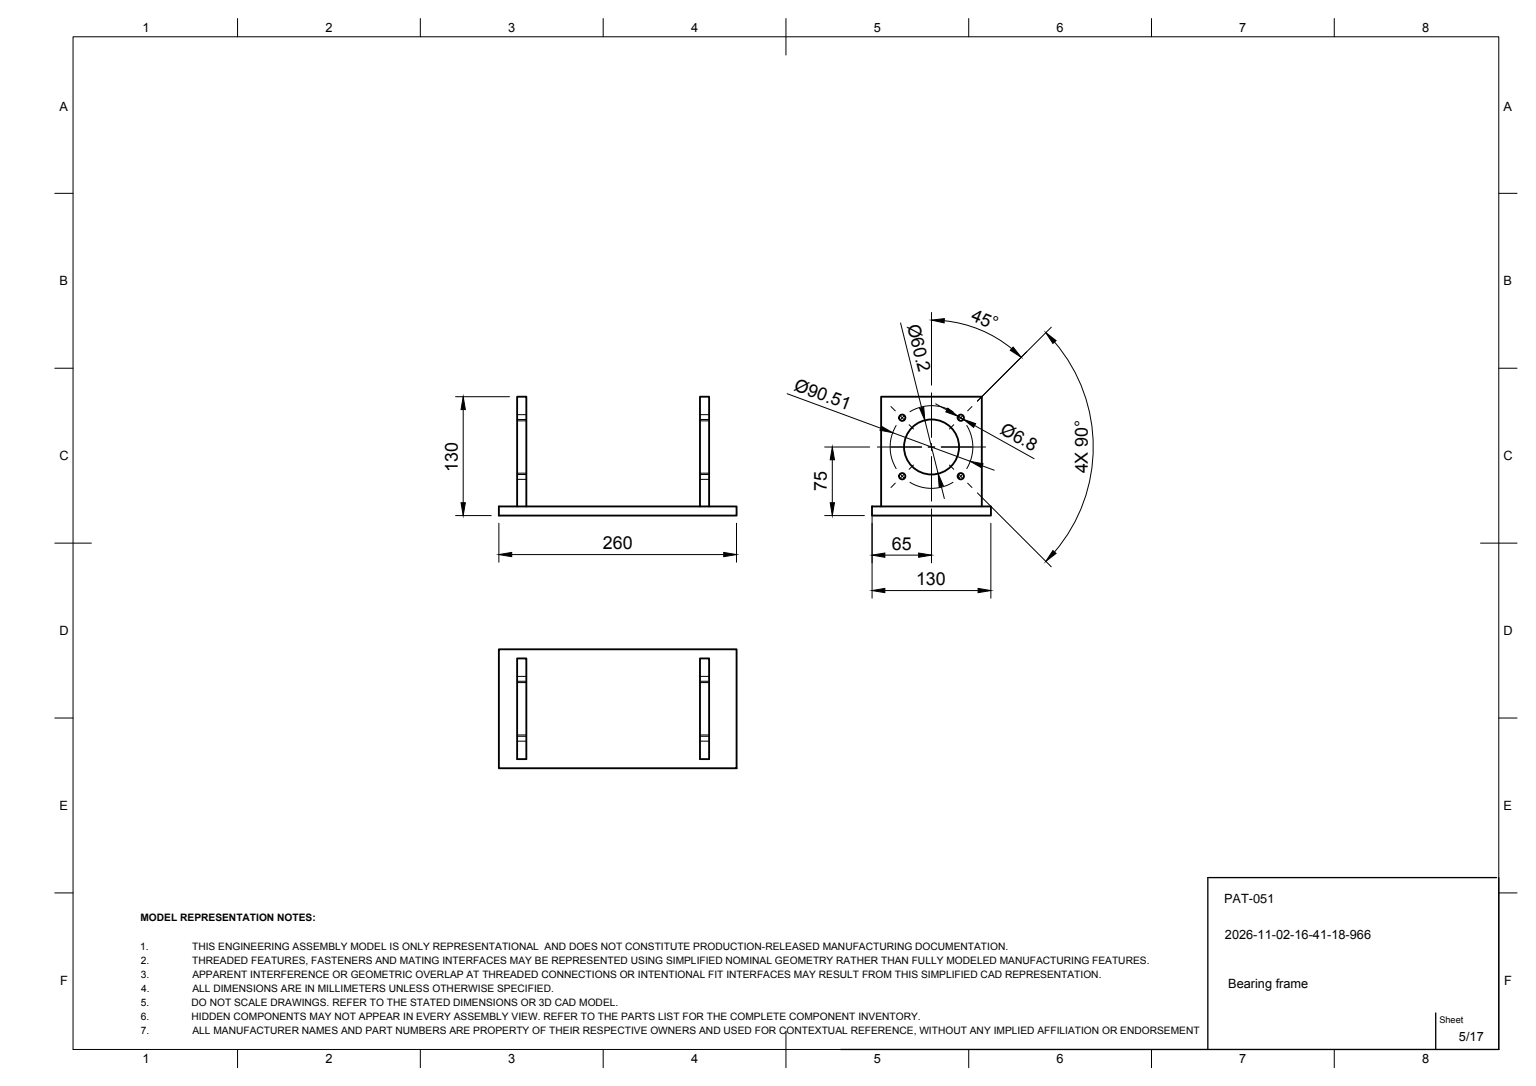
ISO-10303-21;
HEADER;
/* Generated by software containing ST-Developer
 * from STEP Tools, Inc. (www.steptools.com) 
 */

FILE_DESCRIPTION(
/* description */ ('Hand-crank flanged shaft unit'),
/* implementation_level */ '2;1');

FILE_NAME(
/* name */ 'Bearing frame.step',
/* time_stamp */ '2026-10-27T18:35:45-07:00',
/* author */ (''),
/* organization */ (''),
/* preprocessor_version */ 'ST-DEVELOPER v20.2',
/* originating_system */ 'Autodesk Translation Framework v15.17.0.0',
/* authorisation */ '');

FILE_SCHEMA (('AUTOMOTIVE_DESIGN { 1 0 10303 214 3 1 1 }'));
ENDSEC;

DATA;
#10=MECHANICAL_DESIGN_GEOMETRIC_PRESENTATION_REPRESENTATION('',(#279),#6805);
#239=SHAPE_REPRESENTATION_RELATIONSHIP('SRR','None',#6900,#259);
#259=ADVANCED_BREP_SHAPE_REPRESENTATION('',(#300),#6783);
#279=STYLED_ITEM('',(#7091),#300);
#300=MANIFOLD_SOLID_BREP('Body1',#3320);
#320=FACE_BOUND('',#712,.T.);
#321=FACE_BOUND('',#713,.T.);
#322=FACE_BOUND('',#714,.T.);
#323=FACE_BOUND('',#715,.T.);
#324=FACE_BOUND('',#716,.T.);
#325=FACE_BOUND('',#718,.T.);
#326=FACE_BOUND('',#719,.T.);
#327=FACE_BOUND('',#720,.T.);
#328=FACE_BOUND('',#721,.T.);
#329=FACE_BOUND('',#722,.T.);
#330=FACE_BOUND('',#732,.T.);
#331=FACE_BOUND('',#733,.T.);
#332=FACE_BOUND('',#734,.T.);
#333=FACE_BOUND('',#735,.T.);
#334=FACE_BOUND('',#736,.T.);
#335=FACE_BOUND('',#738,.T.);
#336=FACE_BOUND('',#739,.T.);
#337=FACE_BOUND('',#740,.T.);
#338=FACE_BOUND('',#741,.T.);
#339=FACE_BOUND('',#742,.T.);
#340=FACE_BOUND('',#748,.T.);
#341=FACE_BOUND('',#749,.T.);
#410=PLANE('',#3570);
#411=PLANE('',#3571);
#412=PLANE('',#3572);
#413=PLANE('',#3573);
#414=PLANE('',#3574);
#415=PLANE('',#3590);
#416=PLANE('',#3591);
#417=PLANE('',#3592);
#418=PLANE('',#3593);
#419=PLANE('',#3594);
#420=PLANE('',#3595);
#421=PLANE('',#3596);
#422=PLANE('',#3597);
#423=PLANE('',#3598);
#424=PLANE('',#3599);
#425=PLANE('',#3600);
#515=FACE_OUTER_BOUND('',#703,.T.);
#516=FACE_OUTER_BOUND('',#704,.T.);
#517=FACE_OUTER_BOUND('',#705,.T.);
#518=FACE_OUTER_BOUND('',#706,.T.);
#519=FACE_OUTER_BOUND('',#707,.T.);
#520=FACE_OUTER_BOUND('',#708,.T.);
#521=FACE_OUTER_BOUND('',#709,.T.);
#522=FACE_OUTER_BOUND('',#710,.T.);
#523=FACE_OUTER_BOUND('',#711,.T.);
#524=FACE_OUTER_BOUND('',#717,.T.);
#525=FACE_OUTER_BOUND('',#723,.T.);
#526=FACE_OUTER_BOUND('',#724,.T.);
#527=FACE_OUTER_BOUND('',#725,.T.);
#528=FACE_OUTER_BOUND('',#726,.T.);
#529=FACE_OUTER_BOUND('',#727,.T.);
#530=FACE_OUTER_BOUND('',#728,.T.);
#531=FACE_OUTER_BOUND('',#729,.T.);
#532=FACE_OUTER_BOUND('',#730,.T.);
#533=FACE_OUTER_BOUND('',#731,.T.);
#534=FACE_OUTER_BOUND('',#737,.T.);
#535=FACE_OUTER_BOUND('',#743,.T.);
#536=FACE_OUTER_BOUND('',#744,.T.);
#537=FACE_OUTER_BOUND('',#745,.T.);
#538=FACE_OUTER_BOUND('',#746,.T.);
#539=FACE_OUTER_BOUND('',#747,.T.);
#540=FACE_OUTER_BOUND('',#750,.T.);
#703=EDGE_LOOP('',(#2251,#2252,#2253,#2254));
#704=EDGE_LOOP('',(#2255,#2256,#2257,#2258));
#705=EDGE_LOOP('',(#2259,#2260,#2261,#2262));
#706=EDGE_LOOP('',(#2263,#2264,#2265,#2266));
#707=EDGE_LOOP('',(#2267,#2268,#2269,#2270));
#708=EDGE_LOOP('',(#2271,#2272,#2273,#2274));
#709=EDGE_LOOP('',(#2275,#2276,#2277,#2278));
#710=EDGE_LOOP('',(#2279,#2280,#2281,#2282));
#711=EDGE_LOOP('',(#2283,#2284,#2285,#2286));
#712=EDGE_LOOP('',(#2287));
#713=EDGE_LOOP('',(#2288));
#714=EDGE_LOOP('',(#2289));
#715=EDGE_LOOP('',(#2290));
#716=EDGE_LOOP('',(#2291));
#717=EDGE_LOOP('',(#2292,#2293,#2294,#2295));
#718=EDGE_LOOP('',(#2296));
#719=EDGE_LOOP('',(#2297));
#720=EDGE_LOOP('',(#2298));
#721=EDGE_LOOP('',(#2299));
#722=EDGE_LOOP('',(#2300));
#723=EDGE_LOOP('',(#2301,#2302,#2303,#2304));
#724=EDGE_LOOP('',(#2305,#2306,#2307,#2308));
#725=EDGE_LOOP('',(#2309,#2310,#2311,#2312));
#726=EDGE_LOOP('',(#2313,#2314,#2315,#2316));
#727=EDGE_LOOP('',(#2317,#2318,#2319,#2320));
#728=EDGE_LOOP('',(#2321,#2322,#2323,#2324));
#729=EDGE_LOOP('',(#2325,#2326,#2327,#2328));
#730=EDGE_LOOP('',(#2329,#2330,#2331,#2332));
#731=EDGE_LOOP('',(#2333,#2334,#2335,#2336));
#732=EDGE_LOOP('',(#2337));
#733=EDGE_LOOP('',(#2338));
#734=EDGE_LOOP('',(#2339));
#735=EDGE_LOOP('',(#2340));
#736=EDGE_LOOP('',(#2341));
#737=EDGE_LOOP('',(#2342,#2343,#2344,#2345));
#738=EDGE_LOOP('',(#2346));
#739=EDGE_LOOP('',(#2347));
#740=EDGE_LOOP('',(#2348));
#741=EDGE_LOOP('',(#2349));
#742=EDGE_LOOP('',(#2350));
#743=EDGE_LOOP('',(#2351,#2352,#2353,#2354));
#744=EDGE_LOOP('',(#2355,#2356,#2357,#2358));
#745=EDGE_LOOP('',(#2359,#2360,#2361,#2362));
#746=EDGE_LOOP('',(#2363,#2364,#2365,#2366));
#747=EDGE_LOOP('',(#2367,#2368,#2369,#2370));
#748=EDGE_LOOP('',(#2371,#2372,#2373,#2374));
#749=EDGE_LOOP('',(#2375,#2376,#2377,#2378));
#750=EDGE_LOOP('',(#2379,#2380,#2381,#2382));
#981=LINE('',#4939,#1209);
#982=LINE('',#4945,#1210);
#983=LINE('',#4951,#1211);
#984=LINE('',#4957,#1212);
#985=LINE('',#4963,#1213);
#986=LINE('',#4968,#1214);
#987=LINE('',#4970,#1215);
#988=LINE('',#4972,#1216);
#989=LINE('',#4973,#1217);
#990=LINE('',#4977,#1218);
#991=LINE('',#4979,#1219);
#992=LINE('',#4981,#1220);
#993=LINE('',#4982,#1221);
#994=LINE('',#4984,#1222);
#995=LINE('',#4985,#1223);
#996=LINE('',#4987,#1224);
#997=LINE('',#4989,#1225);
#998=LINE('',#4994,#1226);
#999=LINE('',#5000,#1227);
#1000=LINE('',#5006,#1228);
#1001=LINE('',#5012,#1229);
#1002=LINE('',#5018,#1230);
#1003=LINE('',#5023,#1231);
#1004=LINE('',#5025,#1232);
#1005=LINE('',#5027,#1233);
#1006=LINE('',#5028,#1234);
#1007=LINE('',#5032,#1235);
#1008=LINE('',#5034,#1236);
#1009=LINE('',#5036,#1237);
#1010=LINE('',#5037,#1238);
#1011=LINE('',#5039,#1239);
#1012=LINE('',#5040,#1240);
#1013=LINE('',#5042,#1241);
#1014=LINE('',#5044,#1242);
#1015=LINE('',#5048,#1243);
#1016=LINE('',#5050,#1244);
#1017=LINE('',#5052,#1245);
#1018=LINE('',#5053,#1246);
#1019=LINE('',#5056,#1247);
#1020=LINE('',#5058,#1248);
#1021=LINE('',#5059,#1249);
#1022=LINE('',#5062,#1250);
#1023=LINE('',#5064,#1251);
#1024=LINE('',#5065,#1252);
#1025=LINE('',#5067,#1253);
#1026=LINE('',#5068,#1254);
#1209=VECTOR('',#3946,0.34);
#1210=VECTOR('',#3953,0.34);
#1211=VECTOR('',#3960,0.34);
#1212=VECTOR('',#3967,0.34);
#1213=VECTOR('',#3974,3.01);
#1214=VECTOR('',#3979,1.);
#1215=VECTOR('',#3980,1.);
#1216=VECTOR('',#3981,1.);
#1217=VECTOR('',#3982,1.);
#1218=VECTOR('',#3985,1.);
#1219=VECTOR('',#3986,1.);
#1220=VECTOR('',#3987,1.);
#1221=VECTOR('',#3988,1.);
#1222=VECTOR('',#3991,1.);
#1223=VECTOR('',#3992,1.);
#1224=VECTOR('',#3995,1.);
#1225=VECTOR('',#3998,1.);
#1226=VECTOR('',#4003,0.34);
#1227=VECTOR('',#4010,0.34);
#1228=VECTOR('',#4017,0.34);
#1229=VECTOR('',#4024,0.34);
#1230=VECTOR('',#4031,3.01);
#1231=VECTOR('',#4036,1.);
#1232=VECTOR('',#4037,1.);
#1233=VECTOR('',#4038,1.);
#1234=VECTOR('',#4039,1.);
#1235=VECTOR('',#4042,1.);
#1236=VECTOR('',#4043,1.);
#1237=VECTOR('',#4044,1.);
#1238=VECTOR('',#4045,1.);
#1239=VECTOR('',#4048,1.);
#1240=VECTOR('',#4049,1.);
#1241=VECTOR('',#4052,1.);
#1242=VECTOR('',#4055,1.);
#1243=VECTOR('',#4058,1.);
#1244=VECTOR('',#4059,1.);
#1245=VECTOR('',#4060,1.);
#1246=VECTOR('',#4061,1.);
#1247=VECTOR('',#4064,1.);
#1248=VECTOR('',#4065,1.);
#1249=VECTOR('',#4066,1.);
#1250=VECTOR('',#4069,1.);
#1251=VECTOR('',#4070,1.);
#1252=VECTOR('',#4071,1.);
#1253=VECTOR('',#4074,1.);
#1254=VECTOR('',#4075,1.);
#1437=CIRCLE('',#3556,0.34);
#1438=CIRCLE('',#3557,0.34);
#1439=CIRCLE('',#3559,0.34);
#1440=CIRCLE('',#3560,0.34);
#1441=CIRCLE('',#3562,0.34);
#1442=CIRCLE('',#3563,0.34);
#1443=CIRCLE('',#3565,0.34);
#1444=CIRCLE('',#3566,0.34);
#1445=CIRCLE('',#3568,3.01);
#1446=CIRCLE('',#3569,3.01);
#1447=CIRCLE('',#3576,0.34);
#1448=CIRCLE('',#3577,0.34);
#1449=CIRCLE('',#3579,0.34);
#1450=CIRCLE('',#3580,0.34);
#1451=CIRCLE('',#3582,0.34);
#1452=CIRCLE('',#3583,0.34);
#1453=CIRCLE('',#3585,0.34);
#1454=CIRCLE('',#3586,0.34);
#1455=CIRCLE('',#3588,3.01);
#1456=CIRCLE('',#3589,3.01);
#1569=VERTEX_POINT('',#4936);
#1570=VERTEX_POINT('',#4938);
#1571=VERTEX_POINT('',#4942);
#1572=VERTEX_POINT('',#4944);
#1573=VERTEX_POINT('',#4948);
#1574=VERTEX_POINT('',#4950);
#1575=VERTEX_POINT('',#4954);
#1576=VERTEX_POINT('',#4956);
#1577=VERTEX_POINT('',#4960);
#1578=VERTEX_POINT('',#4962);
#1579=VERTEX_POINT('',#4966);
#1580=VERTEX_POINT('',#4967);
#1581=VERTEX_POINT('',#4969);
#1582=VERTEX_POINT('',#4971);
#1583=VERTEX_POINT('',#4975);
#1584=VERTEX_POINT('',#4976);
#1585=VERTEX_POINT('',#4978);
#1586=VERTEX_POINT('',#4980);
#1587=VERTEX_POINT('',#4991);
#1588=VERTEX_POINT('',#4993);
#1589=VERTEX_POINT('',#4997);
#1590=VERTEX_POINT('',#4999);
#1591=VERTEX_POINT('',#5003);
#1592=VERTEX_POINT('',#5005);
#1593=VERTEX_POINT('',#5009);
#1594=VERTEX_POINT('',#5011);
#1595=VERTEX_POINT('',#5015);
#1596=VERTEX_POINT('',#5017);
#1597=VERTEX_POINT('',#5021);
#1598=VERTEX_POINT('',#5022);
#1599=VERTEX_POINT('',#5024);
#1600=VERTEX_POINT('',#5026);
#1601=VERTEX_POINT('',#5030);
#1602=VERTEX_POINT('',#5031);
#1603=VERTEX_POINT('',#5033);
#1604=VERTEX_POINT('',#5035);
#1605=VERTEX_POINT('',#5046);
#1606=VERTEX_POINT('',#5047);
#1607=VERTEX_POINT('',#5049);
#1608=VERTEX_POINT('',#5051);
#1609=VERTEX_POINT('',#5055);
#1610=VERTEX_POINT('',#5057);
#1611=VERTEX_POINT('',#5061);
#1612=VERTEX_POINT('',#5063);
#1843=EDGE_CURVE('',#1569,#1569,#1437,.T.);
#1844=EDGE_CURVE('',#1569,#1570,#981,.T.);
#1845=EDGE_CURVE('',#1570,#1570,#1438,.T.);
#1846=EDGE_CURVE('',#1571,#1571,#1439,.T.);
#1847=EDGE_CURVE('',#1571,#1572,#982,.T.);
#1848=EDGE_CURVE('',#1572,#1572,#1440,.T.);
#1849=EDGE_CURVE('',#1573,#1573,#1441,.T.);
#1850=EDGE_CURVE('',#1573,#1574,#983,.T.);
#1851=EDGE_CURVE('',#1574,#1574,#1442,.T.);
#1852=EDGE_CURVE('',#1575,#1575,#1443,.T.);
#1853=EDGE_CURVE('',#1575,#1576,#984,.T.);
#1854=EDGE_CURVE('',#1576,#1576,#1444,.T.);
#1855=EDGE_CURVE('',#1577,#1577,#1445,.T.);
#1856=EDGE_CURVE('',#1577,#1578,#985,.T.);
#1857=EDGE_CURVE('',#1578,#1578,#1446,.T.);
#1858=EDGE_CURVE('',#1579,#1580,#986,.T.);
#1859=EDGE_CURVE('',#1579,#1581,#987,.T.);
#1860=EDGE_CURVE('',#1582,#1581,#988,.T.);
#1861=EDGE_CURVE('',#1580,#1582,#989,.T.);
#1862=EDGE_CURVE('',#1583,#1584,#990,.T.);
#1863=EDGE_CURVE('',#1585,#1583,#991,.T.);
#1864=EDGE_CURVE('',#1586,#1585,#992,.T.);
#1865=EDGE_CURVE('',#1584,#1586,#993,.T.);
#1866=EDGE_CURVE('',#1584,#1579,#994,.T.);
#1867=EDGE_CURVE('',#1581,#1586,#995,.T.);
#1868=EDGE_CURVE('',#1582,#1585,#996,.T.);
#1869=EDGE_CURVE('',#1583,#1580,#997,.T.);
#1870=EDGE_CURVE('',#1587,#1587,#1447,.T.);
#1871=EDGE_CURVE('',#1587,#1588,#998,.T.);
#1872=EDGE_CURVE('',#1588,#1588,#1448,.T.);
#1873=EDGE_CURVE('',#1589,#1589,#1449,.T.);
#1874=EDGE_CURVE('',#1589,#1590,#999,.T.);
#1875=EDGE_CURVE('',#1590,#1590,#1450,.T.);
#1876=EDGE_CURVE('',#1591,#1591,#1451,.T.);
#1877=EDGE_CURVE('',#1591,#1592,#1000,.T.);
#1878=EDGE_CURVE('',#1592,#1592,#1452,.T.);
#1879=EDGE_CURVE('',#1593,#1593,#1453,.T.);
#1880=EDGE_CURVE('',#1593,#1594,#1001,.T.);
#1881=EDGE_CURVE('',#1594,#1594,#1454,.T.);
#1882=EDGE_CURVE('',#1595,#1595,#1455,.T.);
#1883=EDGE_CURVE('',#1595,#1596,#1002,.T.);
#1884=EDGE_CURVE('',#1596,#1596,#1456,.T.);
#1885=EDGE_CURVE('',#1597,#1598,#1003,.T.);
#1886=EDGE_CURVE('',#1597,#1599,#1004,.T.);
#1887=EDGE_CURVE('',#1600,#1599,#1005,.T.);
#1888=EDGE_CURVE('',#1598,#1600,#1006,.T.);
#1889=EDGE_CURVE('',#1601,#1602,#1007,.T.);
#1890=EDGE_CURVE('',#1603,#1601,#1008,.T.);
#1891=EDGE_CURVE('',#1604,#1603,#1009,.T.);
#1892=EDGE_CURVE('',#1602,#1604,#1010,.T.);
#1893=EDGE_CURVE('',#1602,#1597,#1011,.T.);
#1894=EDGE_CURVE('',#1599,#1604,#1012,.T.);
#1895=EDGE_CURVE('',#1600,#1603,#1013,.T.);
#1896=EDGE_CURVE('',#1601,#1598,#1014,.T.);
#1897=EDGE_CURVE('',#1605,#1606,#1015,.T.);
#1898=EDGE_CURVE('',#1606,#1607,#1016,.T.);
#1899=EDGE_CURVE('',#1608,#1607,#1017,.T.);
#1900=EDGE_CURVE('',#1605,#1608,#1018,.T.);
#1901=EDGE_CURVE('',#1609,#1605,#1019,.T.);
#1902=EDGE_CURVE('',#1610,#1608,#1020,.T.);
#1903=EDGE_CURVE('',#1609,#1610,#1021,.T.);
#1904=EDGE_CURVE('',#1611,#1609,#1022,.T.);
#1905=EDGE_CURVE('',#1612,#1610,#1023,.T.);
#1906=EDGE_CURVE('',#1611,#1612,#1024,.T.);
#1907=EDGE_CURVE('',#1606,#1611,#1025,.T.);
#1908=EDGE_CURVE('',#1607,#1612,#1026,.T.);
#2251=ORIENTED_EDGE('',*,*,#1843,.F.);
#2252=ORIENTED_EDGE('',*,*,#1844,.T.);
#2253=ORIENTED_EDGE('',*,*,#1845,.F.);
#2254=ORIENTED_EDGE('',*,*,#1844,.F.);
#2255=ORIENTED_EDGE('',*,*,#1846,.F.);
#2256=ORIENTED_EDGE('',*,*,#1847,.T.);
#2257=ORIENTED_EDGE('',*,*,#1848,.F.);
#2258=ORIENTED_EDGE('',*,*,#1847,.F.);
#2259=ORIENTED_EDGE('',*,*,#1849,.F.);
#2260=ORIENTED_EDGE('',*,*,#1850,.T.);
#2261=ORIENTED_EDGE('',*,*,#1851,.F.);
#2262=ORIENTED_EDGE('',*,*,#1850,.F.);
#2263=ORIENTED_EDGE('',*,*,#1852,.F.);
#2264=ORIENTED_EDGE('',*,*,#1853,.T.);
#2265=ORIENTED_EDGE('',*,*,#1854,.F.);
#2266=ORIENTED_EDGE('',*,*,#1853,.F.);
#2267=ORIENTED_EDGE('',*,*,#1855,.F.);
#2268=ORIENTED_EDGE('',*,*,#1856,.T.);
#2269=ORIENTED_EDGE('',*,*,#1857,.F.);
#2270=ORIENTED_EDGE('',*,*,#1856,.F.);
#2271=ORIENTED_EDGE('',*,*,#1858,.F.);
#2272=ORIENTED_EDGE('',*,*,#1859,.T.);
#2273=ORIENTED_EDGE('',*,*,#1860,.F.);
#2274=ORIENTED_EDGE('',*,*,#1861,.F.);
#2275=ORIENTED_EDGE('',*,*,#1862,.F.);
#2276=ORIENTED_EDGE('',*,*,#1863,.F.);
#2277=ORIENTED_EDGE('',*,*,#1864,.F.);
#2278=ORIENTED_EDGE('',*,*,#1865,.F.);
#2279=ORIENTED_EDGE('',*,*,#1866,.F.);
#2280=ORIENTED_EDGE('',*,*,#1865,.T.);
#2281=ORIENTED_EDGE('',*,*,#1867,.F.);
#2282=ORIENTED_EDGE('',*,*,#1859,.F.);
#2283=ORIENTED_EDGE('',*,*,#1867,.T.);
#2284=ORIENTED_EDGE('',*,*,#1864,.T.);
#2285=ORIENTED_EDGE('',*,*,#1868,.F.);
#2286=ORIENTED_EDGE('',*,*,#1860,.T.);
#2287=ORIENTED_EDGE('',*,*,#1857,.T.);
#2288=ORIENTED_EDGE('',*,*,#1854,.T.);
#2289=ORIENTED_EDGE('',*,*,#1851,.T.);
#2290=ORIENTED_EDGE('',*,*,#1848,.T.);
#2291=ORIENTED_EDGE('',*,*,#1845,.T.);
#2292=ORIENTED_EDGE('',*,*,#1866,.T.);
#2293=ORIENTED_EDGE('',*,*,#1858,.T.);
#2294=ORIENTED_EDGE('',*,*,#1869,.F.);
#2295=ORIENTED_EDGE('',*,*,#1862,.T.);
#2296=ORIENTED_EDGE('',*,*,#1855,.T.);
#2297=ORIENTED_EDGE('',*,*,#1852,.T.);
#2298=ORIENTED_EDGE('',*,*,#1849,.T.);
#2299=ORIENTED_EDGE('',*,*,#1846,.T.);
#2300=ORIENTED_EDGE('',*,*,#1843,.T.);
#2301=ORIENTED_EDGE('',*,*,#1870,.F.);
#2302=ORIENTED_EDGE('',*,*,#1871,.T.);
#2303=ORIENTED_EDGE('',*,*,#1872,.F.);
#2304=ORIENTED_EDGE('',*,*,#1871,.F.);
#2305=ORIENTED_EDGE('',*,*,#1873,.F.);
#2306=ORIENTED_EDGE('',*,*,#1874,.T.);
#2307=ORIENTED_EDGE('',*,*,#1875,.F.);
#2308=ORIENTED_EDGE('',*,*,#1874,.F.);
#2309=ORIENTED_EDGE('',*,*,#1876,.F.);
#2310=ORIENTED_EDGE('',*,*,#1877,.T.);
#2311=ORIENTED_EDGE('',*,*,#1878,.F.);
#2312=ORIENTED_EDGE('',*,*,#1877,.F.);
#2313=ORIENTED_EDGE('',*,*,#1879,.F.);
#2314=ORIENTED_EDGE('',*,*,#1880,.T.);
#2315=ORIENTED_EDGE('',*,*,#1881,.F.);
#2316=ORIENTED_EDGE('',*,*,#1880,.F.);
#2317=ORIENTED_EDGE('',*,*,#1882,.F.);
#2318=ORIENTED_EDGE('',*,*,#1883,.T.);
#2319=ORIENTED_EDGE('',*,*,#1884,.F.);
#2320=ORIENTED_EDGE('',*,*,#1883,.F.);
#2321=ORIENTED_EDGE('',*,*,#1885,.F.);
#2322=ORIENTED_EDGE('',*,*,#1886,.T.);
#2323=ORIENTED_EDGE('',*,*,#1887,.F.);
#2324=ORIENTED_EDGE('',*,*,#1888,.F.);
#2325=ORIENTED_EDGE('',*,*,#1889,.F.);
#2326=ORIENTED_EDGE('',*,*,#1890,.F.);
#2327=ORIENTED_EDGE('',*,*,#1891,.F.);
#2328=ORIENTED_EDGE('',*,*,#1892,.F.);
#2329=ORIENTED_EDGE('',*,*,#1893,.F.);
#2330=ORIENTED_EDGE('',*,*,#1892,.T.);
#2331=ORIENTED_EDGE('',*,*,#1894,.F.);
#2332=ORIENTED_EDGE('',*,*,#1886,.F.);
#2333=ORIENTED_EDGE('',*,*,#1894,.T.);
#2334=ORIENTED_EDGE('',*,*,#1891,.T.);
#2335=ORIENTED_EDGE('',*,*,#1895,.F.);
#2336=ORIENTED_EDGE('',*,*,#1887,.T.);
#2337=ORIENTED_EDGE('',*,*,#1884,.T.);
#2338=ORIENTED_EDGE('',*,*,#1881,.T.);
#2339=ORIENTED_EDGE('',*,*,#1878,.T.);
#2340=ORIENTED_EDGE('',*,*,#1875,.T.);
#2341=ORIENTED_EDGE('',*,*,#1872,.T.);
#2342=ORIENTED_EDGE('',*,*,#1893,.T.);
#2343=ORIENTED_EDGE('',*,*,#1885,.T.);
#2344=ORIENTED_EDGE('',*,*,#1896,.F.);
#2345=ORIENTED_EDGE('',*,*,#1889,.T.);
#2346=ORIENTED_EDGE('',*,*,#1882,.T.);
#2347=ORIENTED_EDGE('',*,*,#1879,.T.);
#2348=ORIENTED_EDGE('',*,*,#1876,.T.);
#2349=ORIENTED_EDGE('',*,*,#1873,.T.);
#2350=ORIENTED_EDGE('',*,*,#1870,.T.);
#2351=ORIENTED_EDGE('',*,*,#1897,.T.);
#2352=ORIENTED_EDGE('',*,*,#1898,.T.);
#2353=ORIENTED_EDGE('',*,*,#1899,.F.);
#2354=ORIENTED_EDGE('',*,*,#1900,.F.);
#2355=ORIENTED_EDGE('',*,*,#1901,.T.);
#2356=ORIENTED_EDGE('',*,*,#1900,.T.);
#2357=ORIENTED_EDGE('',*,*,#1902,.F.);
#2358=ORIENTED_EDGE('',*,*,#1903,.F.);
#2359=ORIENTED_EDGE('',*,*,#1904,.T.);
#2360=ORIENTED_EDGE('',*,*,#1903,.T.);
#2361=ORIENTED_EDGE('',*,*,#1905,.F.);
#2362=ORIENTED_EDGE('',*,*,#1906,.F.);
#2363=ORIENTED_EDGE('',*,*,#1907,.T.);
#2364=ORIENTED_EDGE('',*,*,#1906,.T.);
#2365=ORIENTED_EDGE('',*,*,#1908,.F.);
#2366=ORIENTED_EDGE('',*,*,#1898,.F.);
#2367=ORIENTED_EDGE('',*,*,#1908,.T.);
#2368=ORIENTED_EDGE('',*,*,#1905,.T.);
#2369=ORIENTED_EDGE('',*,*,#1902,.T.);
#2370=ORIENTED_EDGE('',*,*,#1899,.T.);
#2371=ORIENTED_EDGE('',*,*,#1863,.T.);
#2372=ORIENTED_EDGE('',*,*,#1869,.T.);
#2373=ORIENTED_EDGE('',*,*,#1861,.T.);
#2374=ORIENTED_EDGE('',*,*,#1868,.T.);
#2375=ORIENTED_EDGE('',*,*,#1890,.T.);
#2376=ORIENTED_EDGE('',*,*,#1896,.T.);
#2377=ORIENTED_EDGE('',*,*,#1888,.T.);
#2378=ORIENTED_EDGE('',*,*,#1895,.T.);
#2379=ORIENTED_EDGE('',*,*,#1907,.F.);
#2380=ORIENTED_EDGE('',*,*,#1897,.F.);
#2381=ORIENTED_EDGE('',*,*,#1901,.F.);
#2382=ORIENTED_EDGE('',*,*,#1904,.F.);
#3067=CYLINDRICAL_SURFACE('',#3555,0.34);
#3068=CYLINDRICAL_SURFACE('',#3558,0.34);
#3069=CYLINDRICAL_SURFACE('',#3561,0.34);
#3070=CYLINDRICAL_SURFACE('',#3564,0.34);
#3071=CYLINDRICAL_SURFACE('',#3567,3.01);
#3072=CYLINDRICAL_SURFACE('',#3575,0.34);
#3073=CYLINDRICAL_SURFACE('',#3578,0.34);
#3074=CYLINDRICAL_SURFACE('',#3581,0.34);
#3075=CYLINDRICAL_SURFACE('',#3584,0.34);
#3076=CYLINDRICAL_SURFACE('',#3587,3.01);
#3132=ADVANCED_FACE('',(#515),#3067,.F.);
#3133=ADVANCED_FACE('',(#516),#3068,.F.);
#3134=ADVANCED_FACE('',(#517),#3069,.F.);
#3135=ADVANCED_FACE('',(#518),#3070,.F.);
#3136=ADVANCED_FACE('',(#519),#3071,.F.);
#3137=ADVANCED_FACE('',(#520),#410,.T.);
#3138=ADVANCED_FACE('',(#521),#411,.T.);
#3139=ADVANCED_FACE('',(#522),#412,.T.);
#3140=ADVANCED_FACE('',(#523,#320,#321,#322,#323,#324),#413,.T.);
#3141=ADVANCED_FACE('',(#524,#325,#326,#327,#328,#329),#414,.F.);
#3142=ADVANCED_FACE('',(#525),#3072,.F.);
#3143=ADVANCED_FACE('',(#526),#3073,.F.);
#3144=ADVANCED_FACE('',(#527),#3074,.F.);
#3145=ADVANCED_FACE('',(#528),#3075,.F.);
#3146=ADVANCED_FACE('',(#529),#3076,.F.);
#3147=ADVANCED_FACE('',(#530),#415,.T.);
#3148=ADVANCED_FACE('',(#531),#416,.T.);
#3149=ADVANCED_FACE('',(#532),#417,.T.);
#3150=ADVANCED_FACE('',(#533,#330,#331,#332,#333,#334),#418,.T.);
#3151=ADVANCED_FACE('',(#534,#335,#336,#337,#338,#339),#419,.F.);
#3152=ADVANCED_FACE('',(#535),#420,.T.);
#3153=ADVANCED_FACE('',(#536),#421,.T.);
#3154=ADVANCED_FACE('',(#537),#422,.T.);
#3155=ADVANCED_FACE('',(#538),#423,.T.);
#3156=ADVANCED_FACE('',(#539,#340,#341),#424,.T.);
#3157=ADVANCED_FACE('',(#540),#425,.F.);
#3320=CLOSED_SHELL('',(#3132,#3133,#3134,#3135,#3136,#3137,#3138,#3139,
#3140,#3141,#3142,#3143,#3144,#3145,#3146,#3147,#3148,#3149,#3150,#3151,
#3152,#3153,#3154,#3155,#3156,#3157));
#3554=AXIS2_PLACEMENT_3D('',#4934,#3940,#3941);
#3555=AXIS2_PLACEMENT_3D('',#4935,#3942,#3943);
#3556=AXIS2_PLACEMENT_3D('',#4937,#3944,#3945);
#3557=AXIS2_PLACEMENT_3D('',#4940,#3947,#3948);
#3558=AXIS2_PLACEMENT_3D('',#4941,#3949,#3950);
#3559=AXIS2_PLACEMENT_3D('',#4943,#3951,#3952);
#3560=AXIS2_PLACEMENT_3D('',#4946,#3954,#3955);
#3561=AXIS2_PLACEMENT_3D('',#4947,#3956,#3957);
#3562=AXIS2_PLACEMENT_3D('',#4949,#3958,#3959);
#3563=AXIS2_PLACEMENT_3D('',#4952,#3961,#3962);
#3564=AXIS2_PLACEMENT_3D('',#4953,#3963,#3964);
#3565=AXIS2_PLACEMENT_3D('',#4955,#3965,#3966);
#3566=AXIS2_PLACEMENT_3D('',#4958,#3968,#3969);
#3567=AXIS2_PLACEMENT_3D('',#4959,#3970,#3971);
#3568=AXIS2_PLACEMENT_3D('',#4961,#3972,#3973);
#3569=AXIS2_PLACEMENT_3D('',#4964,#3975,#3976);
#3570=AXIS2_PLACEMENT_3D('',#4965,#3977,#3978);
#3571=AXIS2_PLACEMENT_3D('',#4974,#3983,#3984);
#3572=AXIS2_PLACEMENT_3D('',#4983,#3989,#3990);
#3573=AXIS2_PLACEMENT_3D('',#4986,#3993,#3994);
#3574=AXIS2_PLACEMENT_3D('',#4988,#3996,#3997);
#3575=AXIS2_PLACEMENT_3D('',#4990,#3999,#4000);
#3576=AXIS2_PLACEMENT_3D('',#4992,#4001,#4002);
#3577=AXIS2_PLACEMENT_3D('',#4995,#4004,#4005);
#3578=AXIS2_PLACEMENT_3D('',#4996,#4006,#4007);
#3579=AXIS2_PLACEMENT_3D('',#4998,#4008,#4009);
#3580=AXIS2_PLACEMENT_3D('',#5001,#4011,#4012);
#3581=AXIS2_PLACEMENT_3D('',#5002,#4013,#4014);
#3582=AXIS2_PLACEMENT_3D('',#5004,#4015,#4016);
#3583=AXIS2_PLACEMENT_3D('',#5007,#4018,#4019);
#3584=AXIS2_PLACEMENT_3D('',#5008,#4020,#4021);
#3585=AXIS2_PLACEMENT_3D('',#5010,#4022,#4023);
#3586=AXIS2_PLACEMENT_3D('',#5013,#4025,#4026);
#3587=AXIS2_PLACEMENT_3D('',#5014,#4027,#4028);
#3588=AXIS2_PLACEMENT_3D('',#5016,#4029,#4030);
#3589=AXIS2_PLACEMENT_3D('',#5019,#4032,#4033);
#3590=AXIS2_PLACEMENT_3D('',#5020,#4034,#4035);
#3591=AXIS2_PLACEMENT_3D('',#5029,#4040,#4041);
#3592=AXIS2_PLACEMENT_3D('',#5038,#4046,#4047);
#3593=AXIS2_PLACEMENT_3D('',#5041,#4050,#4051);
#3594=AXIS2_PLACEMENT_3D('',#5043,#4053,#4054);
#3595=AXIS2_PLACEMENT_3D('',#5045,#4056,#4057);
#3596=AXIS2_PLACEMENT_3D('',#5054,#4062,#4063);
#3597=AXIS2_PLACEMENT_3D('',#5060,#4067,#4068);
#3598=AXIS2_PLACEMENT_3D('',#5066,#4072,#4073);
#3599=AXIS2_PLACEMENT_3D('',#5069,#4076,#4077);
#3600=AXIS2_PLACEMENT_3D('',#5070,#4078,#4079);
#3940=DIRECTION('axis',(0.,0.,1.));
#3941=DIRECTION('refdir',(1.,0.,0.));
#3942=DIRECTION('center_axis',(0.,1.,0.));
#3943=DIRECTION('ref_axis',(1.,0.,0.));
#3944=DIRECTION('center_axis',(0.,1.,0.));
#3945=DIRECTION('ref_axis',(1.,0.,0.));
#3946=DIRECTION('',(0.,1.,0.));
#3947=DIRECTION('center_axis',(0.,-1.,0.));
#3948=DIRECTION('ref_axis',(1.,0.,0.));
#3949=DIRECTION('center_axis',(0.,1.,0.));
#3950=DIRECTION('ref_axis',(1.,0.,0.));
#3951=DIRECTION('center_axis',(0.,1.,0.));
#3952=DIRECTION('ref_axis',(1.,0.,0.));
#3953=DIRECTION('',(0.,1.,0.));
#3954=DIRECTION('center_axis',(0.,-1.,0.));
#3955=DIRECTION('ref_axis',(1.,0.,0.));
#3956=DIRECTION('center_axis',(0.,1.,0.));
#3957=DIRECTION('ref_axis',(1.,0.,0.));
#3958=DIRECTION('center_axis',(0.,1.,0.));
#3959=DIRECTION('ref_axis',(1.,0.,0.));
#3960=DIRECTION('',(0.,1.,0.));
#3961=DIRECTION('center_axis',(0.,-1.,0.));
#3962=DIRECTION('ref_axis',(1.,0.,0.));
#3963=DIRECTION('center_axis',(0.,1.,0.));
#3964=DIRECTION('ref_axis',(1.,0.,0.));
#3965=DIRECTION('center_axis',(0.,1.,0.));
#3966=DIRECTION('ref_axis',(1.,0.,0.));
#3967=DIRECTION('',(0.,1.,0.));
#3968=DIRECTION('center_axis',(0.,-1.,0.));
#3969=DIRECTION('ref_axis',(1.,0.,0.));
#3970=DIRECTION('center_axis',(0.,1.,0.));
#3971=DIRECTION('ref_axis',(1.,0.,0.));
#3972=DIRECTION('center_axis',(0.,1.,0.));
#3973=DIRECTION('ref_axis',(1.,0.,0.));
#3974=DIRECTION('',(0.,1.,0.));
#3975=DIRECTION('center_axis',(0.,-1.,0.));
#3976=DIRECTION('ref_axis',(1.,0.,0.));
#3977=DIRECTION('center_axis',(-1.,0.,0.));
#3978=DIRECTION('ref_axis',(0.,0.,1.));
#3979=DIRECTION('',(0.,0.,-1.));
#3980=DIRECTION('',(0.,1.,0.));
#3981=DIRECTION('',(0.,0.,1.));
#3982=DIRECTION('',(0.,1.,0.));
#3983=DIRECTION('center_axis',(1.,0.,0.));
#3984=DIRECTION('ref_axis',(0.,0.,-1.));
#3985=DIRECTION('',(0.,0.,1.));
#3986=DIRECTION('',(0.,-1.,0.));
#3987=DIRECTION('',(0.,0.,-1.));
#3988=DIRECTION('',(0.,1.,0.));
#3989=DIRECTION('center_axis',(0.,0.,1.));
#3990=DIRECTION('ref_axis',(1.,0.,0.));
#3991=DIRECTION('',(-1.,0.,0.));
#3992=DIRECTION('',(1.,0.,0.));
#3993=DIRECTION('center_axis',(0.,1.,0.));
#3994=DIRECTION('ref_axis',(0.,0.,1.));
#3995=DIRECTION('',(1.,0.,0.));
#3996=DIRECTION('center_axis',(0.,1.,0.));
#3997=DIRECTION('ref_axis',(1.,0.,0.));
#3998=DIRECTION('',(-1.,0.,0.));
#3999=DIRECTION('center_axis',(0.,1.,0.));
#4000=DIRECTION('ref_axis',(1.,0.,0.));
#4001=DIRECTION('center_axis',(0.,1.,0.));
#4002=DIRECTION('ref_axis',(1.,0.,0.));
#4003=DIRECTION('',(0.,1.,0.));
#4004=DIRECTION('center_axis',(0.,-1.,0.));
#4005=DIRECTION('ref_axis',(1.,0.,0.));
#4006=DIRECTION('center_axis',(0.,1.,0.));
#4007=DIRECTION('ref_axis',(1.,0.,0.));
#4008=DIRECTION('center_axis',(0.,1.,0.));
#4009=DIRECTION('ref_axis',(1.,0.,0.));
#4010=DIRECTION('',(0.,1.,0.));
#4011=DIRECTION('center_axis',(0.,-1.,0.));
#4012=DIRECTION('ref_axis',(1.,0.,0.));
#4013=DIRECTION('center_axis',(0.,1.,0.));
#4014=DIRECTION('ref_axis',(1.,0.,0.));
#4015=DIRECTION('center_axis',(0.,1.,0.));
#4016=DIRECTION('ref_axis',(1.,0.,0.));
#4017=DIRECTION('',(0.,1.,0.));
#4018=DIRECTION('center_axis',(0.,-1.,0.));
#4019=DIRECTION('ref_axis',(1.,0.,0.));
#4020=DIRECTION('center_axis',(0.,1.,0.));
#4021=DIRECTION('ref_axis',(1.,0.,0.));
#4022=DIRECTION('center_axis',(0.,1.,0.));
#4023=DIRECTION('ref_axis',(1.,0.,0.));
#4024=DIRECTION('',(0.,1.,0.));
#4025=DIRECTION('center_axis',(0.,-1.,0.));
#4026=DIRECTION('ref_axis',(1.,0.,0.));
#4027=DIRECTION('center_axis',(0.,1.,0.));
#4028=DIRECTION('ref_axis',(1.,0.,0.));
#4029=DIRECTION('center_axis',(0.,1.,0.));
#4030=DIRECTION('ref_axis',(1.,0.,0.));
#4031=DIRECTION('',(0.,1.,0.));
#4032=DIRECTION('center_axis',(0.,-1.,0.));
#4033=DIRECTION('ref_axis',(1.,0.,0.));
#4034=DIRECTION('center_axis',(-1.,0.,0.));
#4035=DIRECTION('ref_axis',(0.,0.,1.));
#4036=DIRECTION('',(0.,0.,-1.));
#4037=DIRECTION('',(0.,1.,0.));
#4038=DIRECTION('',(0.,0.,1.));
#4039=DIRECTION('',(0.,1.,0.));
#4040=DIRECTION('center_axis',(1.,0.,0.));
#4041=DIRECTION('ref_axis',(0.,0.,-1.));
#4042=DIRECTION('',(0.,0.,1.));
#4043=DIRECTION('',(0.,-1.,0.));
#4044=DIRECTION('',(0.,0.,-1.));
#4045=DIRECTION('',(0.,1.,0.));
#4046=DIRECTION('center_axis',(0.,0.,1.));
#4047=DIRECTION('ref_axis',(1.,0.,0.));
#4048=DIRECTION('',(-1.,0.,0.));
#4049=DIRECTION('',(1.,0.,0.));
#4050=DIRECTION('center_axis',(0.,1.,0.));
#4051=DIRECTION('ref_axis',(0.,0.,1.));
#4052=DIRECTION('',(1.,0.,0.));
#4053=DIRECTION('center_axis',(0.,1.,0.));
#4054=DIRECTION('ref_axis',(1.,0.,0.));
#4055=DIRECTION('',(-1.,0.,0.));
#4056=DIRECTION('center_axis',(0.,1.,0.));
#4057=DIRECTION('ref_axis',(-1.,0.,0.));
#4058=DIRECTION('',(-1.,0.,0.));
#4059=DIRECTION('',(0.,0.,1.));
#4060=DIRECTION('',(-1.,0.,0.));
#4061=DIRECTION('',(0.,0.,1.));
#4062=DIRECTION('center_axis',(1.,0.,0.));
#4063=DIRECTION('ref_axis',(0.,1.,0.));
#4064=DIRECTION('',(0.,1.,0.));
#4065=DIRECTION('',(0.,1.,0.));
#4066=DIRECTION('',(0.,0.,1.));
#4067=DIRECTION('center_axis',(0.,-1.,0.));
#4068=DIRECTION('ref_axis',(1.,0.,0.));
#4069=DIRECTION('',(1.,0.,0.));
#4070=DIRECTION('',(1.,0.,0.));
#4071=DIRECTION('',(0.,0.,1.));
#4072=DIRECTION('center_axis',(-1.,0.,0.));
#4073=DIRECTION('ref_axis',(0.,-1.,0.));
#4074=DIRECTION('',(0.,-1.,0.));
#4075=DIRECTION('',(0.,-1.,0.));
#4076=DIRECTION('center_axis',(0.,0.,1.));
#4077=DIRECTION('ref_axis',(1.,0.,0.));
#4078=DIRECTION('center_axis',(0.,0.,1.));
#4079=DIRECTION('ref_axis',(1.,0.,0.));
#4934=CARTESIAN_POINT('',(0.,0.,0.));
#4935=CARTESIAN_POINT('Origin',(3.2,19.9,4.3));
#4936=CARTESIAN_POINT('',(2.86,20.,4.3));
#4937=CARTESIAN_POINT('Origin',(3.2,20.,4.3));
#4938=CARTESIAN_POINT('',(2.86,21.,4.3));
#4939=CARTESIAN_POINT('',(2.86,19.9,4.3));
#4940=CARTESIAN_POINT('Origin',(3.2,21.,4.3));
#4941=CARTESIAN_POINT('Origin',(-3.2,19.9,10.7));
#4942=CARTESIAN_POINT('',(-3.54,20.,10.7));
#4943=CARTESIAN_POINT('Origin',(-3.2,20.,10.7));
#4944=CARTESIAN_POINT('',(-3.54,21.,10.7));
#4945=CARTESIAN_POINT('',(-3.54,19.9,10.7));
#4946=CARTESIAN_POINT('Origin',(-3.2,21.,10.7));
#4947=CARTESIAN_POINT('Origin',(-3.2,19.9,4.3));
#4948=CARTESIAN_POINT('',(-3.54,20.,4.3));
#4949=CARTESIAN_POINT('Origin',(-3.2,20.,4.3));
#4950=CARTESIAN_POINT('',(-3.54,21.,4.3));
#4951=CARTESIAN_POINT('',(-3.54,19.9,4.3));
#4952=CARTESIAN_POINT('Origin',(-3.2,21.,4.3));
#4953=CARTESIAN_POINT('Origin',(3.2,19.9,10.7));
#4954=CARTESIAN_POINT('',(2.86,20.,10.7));
#4955=CARTESIAN_POINT('Origin',(3.2,20.,10.7));
#4956=CARTESIAN_POINT('',(2.86,21.,10.7));
#4957=CARTESIAN_POINT('',(2.86,19.9,10.7));
#4958=CARTESIAN_POINT('Origin',(3.2,21.,10.7));
#4959=CARTESIAN_POINT('Origin',(0.,19.9,7.5));
#4960=CARTESIAN_POINT('',(-3.01,20.,7.5));
#4961=CARTESIAN_POINT('Origin',(0.,20.,7.5));
#4962=CARTESIAN_POINT('',(-3.01,21.,7.5));
#4963=CARTESIAN_POINT('',(-3.01,19.9,7.5));
#4964=CARTESIAN_POINT('Origin',(0.,21.,7.5));
#4965=CARTESIAN_POINT('Origin',(-5.5,20.,1.));
#4966=CARTESIAN_POINT('',(-5.5,20.,13.));
#4967=CARTESIAN_POINT('',(-5.5,20.,1.));
#4968=CARTESIAN_POINT('',(-5.5,20.,13.));
#4969=CARTESIAN_POINT('',(-5.5,21.,13.));
#4970=CARTESIAN_POINT('',(-5.5,20.,13.));
#4971=CARTESIAN_POINT('',(-5.5,21.,1.));
#4972=CARTESIAN_POINT('',(-5.5,21.,13.));
#4973=CARTESIAN_POINT('',(-5.5,15.,1.));
#4974=CARTESIAN_POINT('Origin',(5.5,20.,13.));
#4975=CARTESIAN_POINT('',(5.5,20.,1.));
#4976=CARTESIAN_POINT('',(5.5,20.,13.));
#4977=CARTESIAN_POINT('',(5.5,20.,1.));
#4978=CARTESIAN_POINT('',(5.5,21.,1.));
#4979=CARTESIAN_POINT('',(5.5,15.,1.));
#4980=CARTESIAN_POINT('',(5.5,21.,13.));
#4981=CARTESIAN_POINT('',(5.5,21.,1.));
#4982=CARTESIAN_POINT('',(5.5,20.,13.));
#4983=CARTESIAN_POINT('Origin',(-5.5,20.,13.));
#4984=CARTESIAN_POINT('',(5.5,20.,13.));
#4985=CARTESIAN_POINT('',(5.5,21.,13.));
#4986=CARTESIAN_POINT('Origin',(0.,21.,7.));
#4987=CARTESIAN_POINT('',(0.,21.,1.));
#4988=CARTESIAN_POINT('Origin',(0.,20.,7.));
#4989=CARTESIAN_POINT('',(0.,20.,1.));
#4990=CARTESIAN_POINT('Origin',(3.2,-0.1,4.3));
#4991=CARTESIAN_POINT('',(2.86,0.,4.3));
#4992=CARTESIAN_POINT('Origin',(3.2,0.,4.3));
#4993=CARTESIAN_POINT('',(2.86,1.,4.3));
#4994=CARTESIAN_POINT('',(2.86,-0.1,4.3));
#4995=CARTESIAN_POINT('Origin',(3.2,1.,4.3));
#4996=CARTESIAN_POINT('Origin',(-3.2,-0.1,10.7));
#4997=CARTESIAN_POINT('',(-3.54,0.,10.7));
#4998=CARTESIAN_POINT('Origin',(-3.2,0.,10.7));
#4999=CARTESIAN_POINT('',(-3.54,1.,10.7));
#5000=CARTESIAN_POINT('',(-3.54,-0.1,10.7));
#5001=CARTESIAN_POINT('Origin',(-3.2,1.,10.7));
#5002=CARTESIAN_POINT('Origin',(-3.2,-0.1,4.3));
#5003=CARTESIAN_POINT('',(-3.54,0.,4.3));
#5004=CARTESIAN_POINT('Origin',(-3.2,0.,4.3));
#5005=CARTESIAN_POINT('',(-3.54,1.,4.3));
#5006=CARTESIAN_POINT('',(-3.54,-0.1,4.3));
#5007=CARTESIAN_POINT('Origin',(-3.2,1.,4.3));
#5008=CARTESIAN_POINT('Origin',(3.2,-0.1,10.7));
#5009=CARTESIAN_POINT('',(2.86,0.,10.7));
#5010=CARTESIAN_POINT('Origin',(3.2,0.,10.7));
#5011=CARTESIAN_POINT('',(2.86,1.,10.7));
#5012=CARTESIAN_POINT('',(2.86,-0.1,10.7));
#5013=CARTESIAN_POINT('Origin',(3.2,1.,10.7));
#5014=CARTESIAN_POINT('Origin',(0.,-0.1,7.5));
#5015=CARTESIAN_POINT('',(-3.01,0.,7.5));
#5016=CARTESIAN_POINT('Origin',(0.,0.,7.5));
#5017=CARTESIAN_POINT('',(-3.01,1.,7.5));
#5018=CARTESIAN_POINT('',(-3.01,-0.1,7.5));
#5019=CARTESIAN_POINT('Origin',(0.,1.,7.5));
#5020=CARTESIAN_POINT('Origin',(-5.5,0.,1.));
#5021=CARTESIAN_POINT('',(-5.5,0.,13.));
#5022=CARTESIAN_POINT('',(-5.5,0.,1.));
#5023=CARTESIAN_POINT('',(-5.5,0.,13.));
#5024=CARTESIAN_POINT('',(-5.5,1.,13.));
#5025=CARTESIAN_POINT('',(-5.5,0.,13.));
#5026=CARTESIAN_POINT('',(-5.5,1.,1.));
#5027=CARTESIAN_POINT('',(-5.5,1.,13.));
#5028=CARTESIAN_POINT('',(-5.5,5.,1.));
#5029=CARTESIAN_POINT('Origin',(5.5,0.,13.));
#5030=CARTESIAN_POINT('',(5.5,0.,1.));
#5031=CARTESIAN_POINT('',(5.5,0.,13.));
#5032=CARTESIAN_POINT('',(5.5,0.,1.));
#5033=CARTESIAN_POINT('',(5.5,1.,1.));
#5034=CARTESIAN_POINT('',(5.5,5.,1.));
#5035=CARTESIAN_POINT('',(5.5,1.,13.));
#5036=CARTESIAN_POINT('',(5.5,1.,1.));
#5037=CARTESIAN_POINT('',(5.5,0.,13.));
#5038=CARTESIAN_POINT('Origin',(-5.5,0.,13.));
#5039=CARTESIAN_POINT('',(5.5,0.,13.));
#5040=CARTESIAN_POINT('',(5.5,1.,13.));
#5041=CARTESIAN_POINT('Origin',(0.,1.,7.));
#5042=CARTESIAN_POINT('',(0.,1.,1.));
#5043=CARTESIAN_POINT('Origin',(0.,0.,7.));
#5044=CARTESIAN_POINT('',(0.,0.,1.));
#5045=CARTESIAN_POINT('Origin',(6.5,23.,0.));
#5046=CARTESIAN_POINT('',(6.5,23.,0.));
#5047=CARTESIAN_POINT('',(-6.5,23.,0.));
#5048=CARTESIAN_POINT('',(6.5,23.,0.));
#5049=CARTESIAN_POINT('',(-6.5,23.,1.));
#5050=CARTESIAN_POINT('',(-6.5,23.,0.));
#5051=CARTESIAN_POINT('',(6.5,23.,1.));
#5052=CARTESIAN_POINT('',(6.5,23.,1.));
#5053=CARTESIAN_POINT('',(6.5,23.,0.));
#5054=CARTESIAN_POINT('Origin',(6.5,-3.,0.));
#5055=CARTESIAN_POINT('',(6.5,-3.,0.));
#5056=CARTESIAN_POINT('',(6.5,-3.,0.));
#5057=CARTESIAN_POINT('',(6.5,-3.,1.));
#5058=CARTESIAN_POINT('',(6.5,-3.,1.));
#5059=CARTESIAN_POINT('',(6.5,-3.,0.));
#5060=CARTESIAN_POINT('Origin',(-6.5,-3.,0.));
#5061=CARTESIAN_POINT('',(-6.5,-3.,0.));
#5062=CARTESIAN_POINT('',(-6.5,-3.,0.));
#5063=CARTESIAN_POINT('',(-6.5,-3.,1.));
#5064=CARTESIAN_POINT('',(-6.5,-3.,1.));
#5065=CARTESIAN_POINT('',(-6.5,-3.,0.));
#5066=CARTESIAN_POINT('Origin',(-6.5,23.,0.));
#5067=CARTESIAN_POINT('',(-6.5,23.,0.));
#5068=CARTESIAN_POINT('',(-6.5,23.,1.));
#5069=CARTESIAN_POINT('Origin',(0.,10.,1.));
#5070=CARTESIAN_POINT('Origin',(0.,10.,0.));
#6758=UNCERTAINTY_MEASURE_WITH_UNIT(LENGTH_MEASURE(0.001),#6806,
'DISTANCE_ACCURACY_VALUE',
'Maximum model space distance between geometric entities at asserted c
onnectivities');
#6780=UNCERTAINTY_MEASURE_WITH_UNIT(LENGTH_MEASURE(0.001),#6806,
'DISTANCE_ACCURACY_VALUE',
'Maximum model space distance between geometric entities at asserted c
onnectivities');
#6783=(
GEOMETRIC_REPRESENTATION_CONTEXT(3)
GLOBAL_UNCERTAINTY_ASSIGNED_CONTEXT((#6758))
GLOBAL_UNIT_ASSIGNED_CONTEXT((#6806,#6808,#6809))
REPRESENTATION_CONTEXT('','3D')
);
#6805=(
GEOMETRIC_REPRESENTATION_CONTEXT(3)
GLOBAL_UNCERTAINTY_ASSIGNED_CONTEXT((#6780))
GLOBAL_UNIT_ASSIGNED_CONTEXT((#6806,#6808,#6809))
REPRESENTATION_CONTEXT('','3D')
);
#6806=(
LENGTH_UNIT()
NAMED_UNIT(*)
SI_UNIT(.CENTI.,.METRE.)
);
#6808=(
NAMED_UNIT(*)
PLANE_ANGLE_UNIT()
SI_UNIT($,.RADIAN.)
);
#6809=(
NAMED_UNIT(*)
SI_UNIT($,.STERADIAN.)
SOLID_ANGLE_UNIT()
);
#6812=SHAPE_DEFINITION_REPRESENTATION(#6836,#6900);
#6836=PRODUCT_DEFINITION_SHAPE('',$,#6925);
#6900=SHAPE_REPRESENTATION('',(#3554),#6783);
#6922=PRODUCT_DEFINITION_CONTEXT('part definition',#6996,'design');
#6925=PRODUCT_DEFINITION('Bearing frame','Bearing frame',#6949,#6922);
#6949=PRODUCT_DEFINITION_FORMATION('',$,#7000);
#6996=APPLICATION_CONTEXT(
'Core Data for Automotive Mechanical Design Process');
#6997=PRODUCT_CONTEXT('part definition',#6996,'mechanical');
#7000=PRODUCT('Bearing frame','Bearing frame','Bearing frame',(#6997));
#7085=COLOUR_RGB('Grey',0.48,0.52,0.57);
#7086=FILL_AREA_STYLE_COLOUR('',#7085);
#7087=FILL_AREA_STYLE('',(#7086));
#7088=SURFACE_STYLE_FILL_AREA(#7087);
#7089=SURFACE_SIDE_STYLE('',(#7088));
#7090=SURFACE_STYLE_USAGE(.BOTH.,#7089);
#7091=PRESENTATION_STYLE_ASSIGNMENT((#7090));
ENDSEC;
END-ISO-10303-21;
